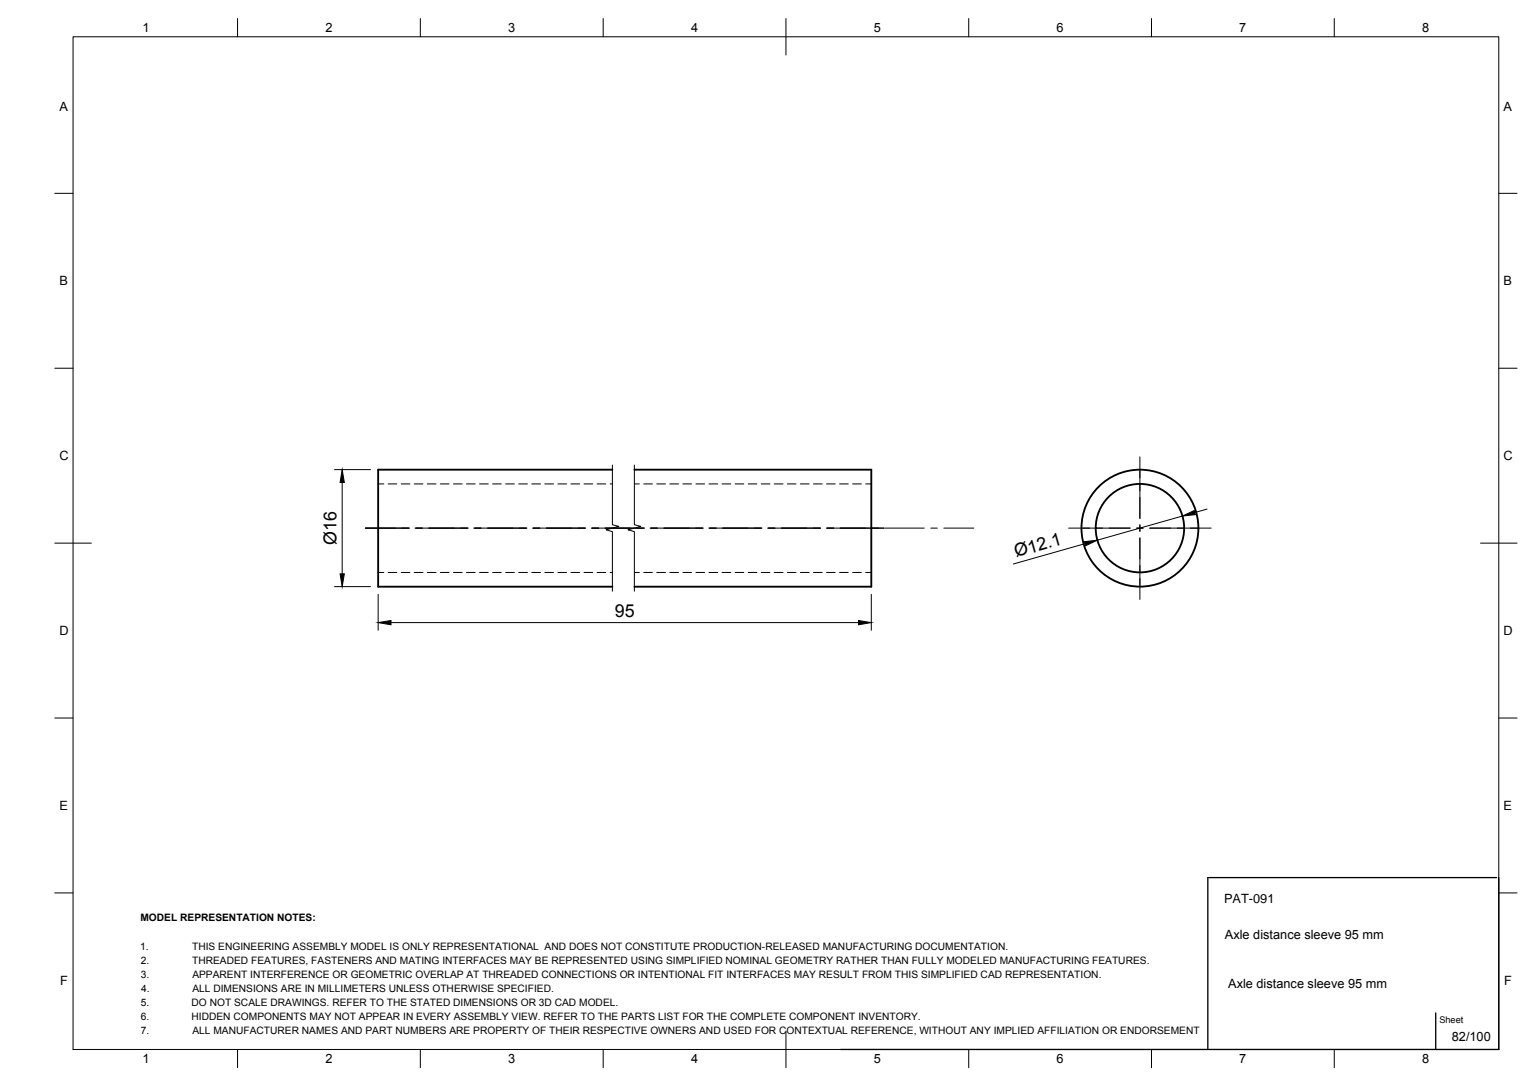
ISO-10303-21;
HEADER;
/* Generated by software containing ST-Developer
 * from STEP Tools, Inc. (www.steptools.com) 
 */

FILE_DESCRIPTION(
/* description */ ('PAT-091'),
/* implementation_level */ '2;1');

FILE_NAME(
/* name */ 'Axle distance sleeve 95 mm.step',
/* time_stamp */ '2026-10-27T15:34:44-07:00',
/* author */ (''),
/* organization */ (''),
/* preprocessor_version */ 'ST-DEVELOPER v20.2',
/* originating_system */ 'Autodesk Translation Framework v15.17.0.0',
/* authorisation */ '');

FILE_SCHEMA (('AUTOMOTIVE_DESIGN { 1 0 10303 214 3 1 1 }'));
ENDSEC;

DATA;
#10=MECHANICAL_DESIGN_GEOMETRIC_PRESENTATION_REPRESENTATION('',(#1040),#25100);
#820=SHAPE_REPRESENTATION_RELATIONSHIP('SRR','None',#25586,#930);
#930=ADVANCED_BREP_SHAPE_REPRESENTATION('',(#1162),#25056);
#1040=STYLED_ITEM('',(#26191),#1162);
#1162=MANIFOLD_SOLID_BREP('Body1',#13319);
#1518=FACE_BOUND('',#3708,.T.);
#1519=FACE_BOUND('',#3710,.T.);
#1931=PLANE('',#15653);
#1932=PLANE('',#15654);
#2584=FACE_OUTER_BOUND('',#3705,.T.);
#2585=FACE_OUTER_BOUND('',#3706,.T.);
#2586=FACE_OUTER_BOUND('',#3707,.T.);
#2587=FACE_OUTER_BOUND('',#3709,.T.);
#3705=EDGE_LOOP('',(#11044,#11045,#11046,#11047));
#3706=EDGE_LOOP('',(#11048,#11049,#11050,#11051));
#3707=EDGE_LOOP('',(#11052));
#3708=EDGE_LOOP('',(#11053));
#3709=EDGE_LOOP('',(#11054));
#3710=EDGE_LOOP('',(#11055));
#4694=LINE('',#23354,#5434);
#4695=LINE('',#23360,#5435);
#5434=VECTOR('',#19166,0.605);
#5435=VECTOR('',#19173,0.800000000000001);
#6066=CIRCLE('',#15648,0.605);
#6067=CIRCLE('',#15649,0.605);
#6068=CIRCLE('',#15651,0.800000000000001);
#6069=CIRCLE('',#15652,0.800000000000001);
#7071=VERTEX_POINT('',#23351);
#7072=VERTEX_POINT('',#23353);
#7073=VERTEX_POINT('',#23357);
#7074=VERTEX_POINT('',#23359);
#8457=EDGE_CURVE('',#7071,#7071,#6066,.T.);
#8458=EDGE_CURVE('',#7071,#7072,#4694,.T.);
#8459=EDGE_CURVE('',#7072,#7072,#6067,.T.);
#8460=EDGE_CURVE('',#7073,#7073,#6068,.T.);
#8461=EDGE_CURVE('',#7073,#7074,#4695,.T.);
#8462=EDGE_CURVE('',#7074,#7074,#6069,.T.);
#11044=ORIENTED_EDGE('',*,*,#8457,.F.);
#11045=ORIENTED_EDGE('',*,*,#8458,.T.);
#11046=ORIENTED_EDGE('',*,*,#8459,.T.);
#11047=ORIENTED_EDGE('',*,*,#8458,.F.);
#11048=ORIENTED_EDGE('',*,*,#8460,.F.);
#11049=ORIENTED_EDGE('',*,*,#8461,.T.);
#11050=ORIENTED_EDGE('',*,*,#8462,.T.);
#11051=ORIENTED_EDGE('',*,*,#8461,.F.);
#11052=ORIENTED_EDGE('',*,*,#8460,.T.);
#11053=ORIENTED_EDGE('',*,*,#8457,.T.);
#11054=ORIENTED_EDGE('',*,*,#8462,.F.);
#11055=ORIENTED_EDGE('',*,*,#8459,.F.);
#12296=CYLINDRICAL_SURFACE('',#15647,0.605);
#12297=CYLINDRICAL_SURFACE('',#15650,0.800000000000001);
#12951=ADVANCED_FACE('',(#2584),#12296,.F.);
#12952=ADVANCED_FACE('',(#2585),#12297,.T.);
#12953=ADVANCED_FACE('',(#2586,#1518),#1931,.T.);
#12954=ADVANCED_FACE('',(#2587,#1519),#1932,.F.);
#13319=CLOSED_SHELL('',(#12951,#12952,#12953,#12954));
#15646=AXIS2_PLACEMENT_3D('',#23349,#19160,#19161);
#15647=AXIS2_PLACEMENT_3D('',#23350,#19162,#19163);
#15648=AXIS2_PLACEMENT_3D('',#23352,#19164,#19165);
#15649=AXIS2_PLACEMENT_3D('',#23355,#19167,#19168);
#15650=AXIS2_PLACEMENT_3D('',#23356,#19169,#19170);
#15651=AXIS2_PLACEMENT_3D('',#23358,#19171,#19172);
#15652=AXIS2_PLACEMENT_3D('',#23361,#19174,#19175);
#15653=AXIS2_PLACEMENT_3D('',#23362,#19176,#19177);
#15654=AXIS2_PLACEMENT_3D('',#23363,#19178,#19179);
#19160=DIRECTION('axis',(0.,0.,1.));
#19161=DIRECTION('refdir',(1.,0.,0.));
#19162=DIRECTION('center_axis',(0.,1.,0.));
#19163=DIRECTION('ref_axis',(1.,0.,0.));
#19164=DIRECTION('center_axis',(0.,-1.,0.));
#19165=DIRECTION('ref_axis',(1.,0.,0.));
#19166=DIRECTION('',(0.,-1.,0.));
#19167=DIRECTION('center_axis',(0.,-1.,0.));
#19168=DIRECTION('ref_axis',(1.,0.,0.));
#19169=DIRECTION('center_axis',(0.,1.,0.));
#19170=DIRECTION('ref_axis',(1.,0.,0.));
#19171=DIRECTION('center_axis',(0.,1.,0.));
#19172=DIRECTION('ref_axis',(1.,0.,0.));
#19173=DIRECTION('',(0.,-1.,0.));
#19174=DIRECTION('center_axis',(0.,1.,0.));
#19175=DIRECTION('ref_axis',(1.,0.,0.));
#19176=DIRECTION('center_axis',(0.,1.,0.));
#19177=DIRECTION('ref_axis',(1.,0.,0.));
#19178=DIRECTION('center_axis',(0.,1.,0.));
#19179=DIRECTION('ref_axis',(1.,0.,0.));
#23349=CARTESIAN_POINT('',(0.,0.,0.));
#23350=CARTESIAN_POINT('Origin',(19.3649167310371,-4.5,8.));
#23351=CARTESIAN_POINT('',(18.7599167310371,5.,8.));
#23352=CARTESIAN_POINT('Origin',(19.3649167310371,5.,8.));
#23353=CARTESIAN_POINT('',(18.7599167310371,-4.5,8.));
#23354=CARTESIAN_POINT('',(18.7599167310371,-4.5,8.));
#23355=CARTESIAN_POINT('Origin',(19.3649167310371,-4.5,8.));
#23356=CARTESIAN_POINT('Origin',(19.3649167310371,-4.5,8.));
#23357=CARTESIAN_POINT('',(18.5649167310371,5.,8.));
#23358=CARTESIAN_POINT('Origin',(19.3649167310371,5.,8.));
#23359=CARTESIAN_POINT('',(18.5649167310371,-4.5,8.));
#23360=CARTESIAN_POINT('',(18.5649167310371,-4.5,8.));
#23361=CARTESIAN_POINT('Origin',(19.3649167310371,-4.5,8.));
#23362=CARTESIAN_POINT('Origin',(19.3649167310371,5.,8.));
#23363=CARTESIAN_POINT('Origin',(19.3649167310371,-4.5,8.));
#24935=UNCERTAINTY_MEASURE_WITH_UNIT(LENGTH_MEASURE(0.001),#25101,
'DISTANCE_ACCURACY_VALUE',
'Maximum model space distance between geometric entities at asserted c
onnectivities');
#24979=UNCERTAINTY_MEASURE_WITH_UNIT(LENGTH_MEASURE(0.001),#25101,
'DISTANCE_ACCURACY_VALUE',
'Maximum model space distance between geometric entities at asserted c
onnectivities');
#25056=(
GEOMETRIC_REPRESENTATION_CONTEXT(3)
GLOBAL_UNCERTAINTY_ASSIGNED_CONTEXT((#24935))
GLOBAL_UNIT_ASSIGNED_CONTEXT((#25101,#25103,#25104))
REPRESENTATION_CONTEXT('','3D')
);
#25100=(
GEOMETRIC_REPRESENTATION_CONTEXT(3)
GLOBAL_UNCERTAINTY_ASSIGNED_CONTEXT((#24979))
GLOBAL_UNIT_ASSIGNED_CONTEXT((#25101,#25103,#25104))
REPRESENTATION_CONTEXT('','3D')
);
#25101=(
LENGTH_UNIT()
NAMED_UNIT(*)
SI_UNIT(.CENTI.,.METRE.)
);
#25103=(
NAMED_UNIT(*)
PLANE_ANGLE_UNIT()
SI_UNIT($,.RADIAN.)
);
#25104=(
NAMED_UNIT(*)
SI_UNIT($,.STERADIAN.)
SOLID_ANGLE_UNIT()
);
#25181=SHAPE_DEFINITION_REPRESENTATION(#25303,#25586);
#25303=PRODUCT_DEFINITION_SHAPE('',$,#25707);
#25586=SHAPE_REPRESENTATION('',(#15646),#25056);
#25630=PRODUCT_DEFINITION_CONTEXT('part definition',#25992,'design');
#25707=PRODUCT_DEFINITION('Axle distance sleeve 95 mm',
'Axle distance sleeve 95 mm',#25827,#25630);
#25827=PRODUCT_DEFINITION_FORMATION('',$,#26070);
#25992=APPLICATION_CONTEXT(
'Core Data for Automotive Mechanical Design Process');
#25993=PRODUCT_CONTEXT('part definition',#25992,'mechanical');
#26070=PRODUCT('Axle distance sleeve 95 mm',
'Axle distance sleeve 95 mm','Axle distance sleeve 95 mm',(#25993));
#26185=COLOUR_RGB('Grey',0.48,0.52,0.57);
#26186=FILL_AREA_STYLE_COLOUR('',#26185);
#26187=FILL_AREA_STYLE('',(#26186));
#26188=SURFACE_STYLE_FILL_AREA(#26187);
#26189=SURFACE_SIDE_STYLE('',(#26188));
#26190=SURFACE_STYLE_USAGE(.BOTH.,#26189);
#26191=PRESENTATION_STYLE_ASSIGNMENT((#26190));
ENDSEC;
END-ISO-10303-21;
